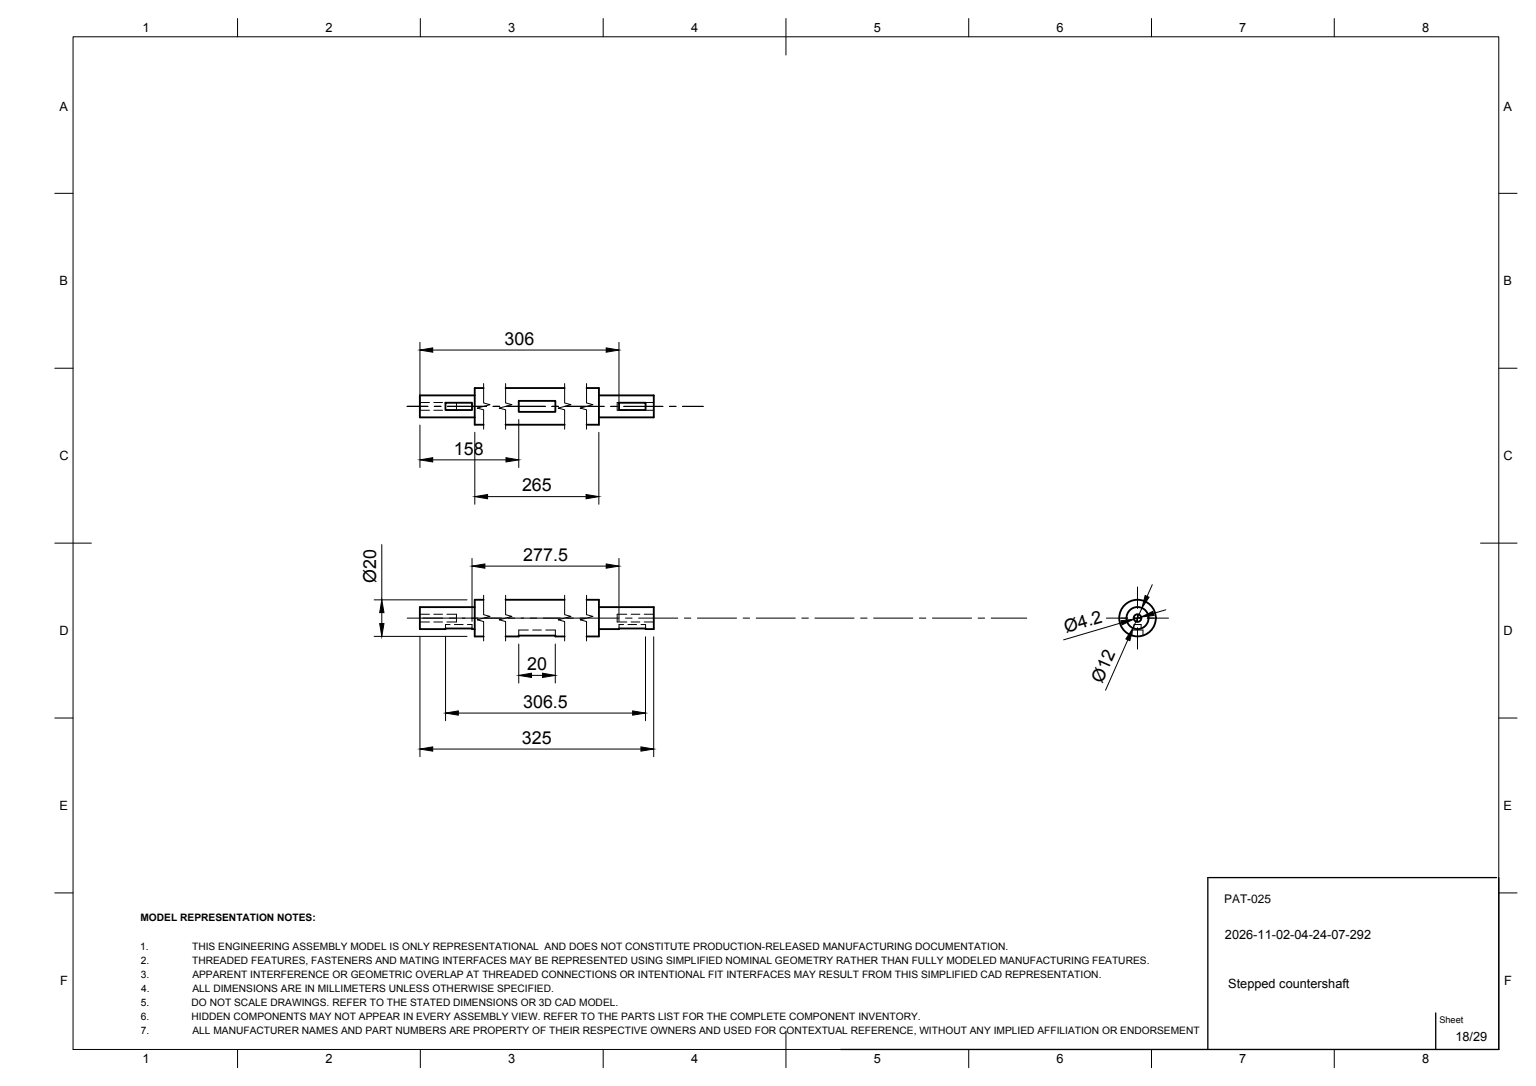
ISO-10303-21;
HEADER;
/* Generated by software containing ST-Developer
 * from STEP Tools, Inc. (www.steptools.com) 
 */

FILE_DESCRIPTION(
/* description */ ('Counter shaft with two pulleys and keyed hub'),
/* implementation_level */ '2;1');

FILE_NAME(
/* name */ 'Stepped countershaft.step',
/* time_stamp */ '2026-10-27T10:46:10-07:00',
/* author */ (''),
/* organization */ (''),
/* preprocessor_version */ 'ST-DEVELOPER v20.2',
/* originating_system */ 'Autodesk Translation Framework v15.17.0.0',
/* authorisation */ '');

FILE_SCHEMA (('AUTOMOTIVE_DESIGN { 1 0 10303 214 3 1 1 }'));
ENDSEC;

DATA;
#10=MECHANICAL_DESIGN_GEOMETRIC_PRESENTATION_REPRESENTATION('',(#302),#10821);
#251=SHAPE_REPRESENTATION_RELATIONSHIP('SRR','None',#10939,#276);
#276=ADVANCED_BREP_SHAPE_REPRESENTATION('',(#327),#10807);
#302=STYLED_ITEM('',(#11135),#327);
#327=MANIFOLD_SOLID_BREP('Body1',#5586);
#388=FACE_BOUND('',#1069,.T.);
#389=FACE_BOUND('',#1071,.T.);
#390=FACE_BOUND('',#1073,.T.);
#391=FACE_BOUND('',#1075,.T.);
#392=FACE_BOUND('',#1077,.T.);
#393=FACE_BOUND('',#1079,.T.);
#394=FACE_BOUND('',#1081,.T.);
#494=PLANE('',#6072);
#495=PLANE('',#6073);
#496=PLANE('',#6075);
#497=PLANE('',#6076);
#498=PLANE('',#6077);
#499=PLANE('',#6082);
#500=PLANE('',#6086);
#501=PLANE('',#6087);
#502=PLANE('',#6088);
#503=PLANE('',#6090);
#504=PLANE('',#6091);
#505=PLANE('',#6092);
#506=PLANE('',#6094);
#507=PLANE('',#6095);
#508=PLANE('',#6097);
#509=PLANE('',#6098);
#510=PLANE('',#6099);
#511=PLANE('',#6104);
#512=PLANE('',#6108);
#513=PLANE('',#6112);
#514=PLANE('',#6113);
#687=FACE_OUTER_BOUND('',#1049,.T.);
#688=FACE_OUTER_BOUND('',#1050,.T.);
#689=FACE_OUTER_BOUND('',#1051,.T.);
#690=FACE_OUTER_BOUND('',#1052,.T.);
#691=FACE_OUTER_BOUND('',#1053,.T.);
#692=FACE_OUTER_BOUND('',#1054,.T.);
#693=FACE_OUTER_BOUND('',#1055,.T.);
#694=FACE_OUTER_BOUND('',#1056,.T.);
#695=FACE_OUTER_BOUND('',#1057,.T.);
#696=FACE_OUTER_BOUND('',#1058,.T.);
#697=FACE_OUTER_BOUND('',#1059,.T.);
#698=FACE_OUTER_BOUND('',#1060,.T.);
#699=FACE_OUTER_BOUND('',#1061,.T.);
#700=FACE_OUTER_BOUND('',#1062,.T.);
#701=FACE_OUTER_BOUND('',#1063,.T.);
#702=FACE_OUTER_BOUND('',#1064,.T.);
#703=FACE_OUTER_BOUND('',#1065,.T.);
#704=FACE_OUTER_BOUND('',#1066,.T.);
#705=FACE_OUTER_BOUND('',#1067,.T.);
#706=FACE_OUTER_BOUND('',#1068,.T.);
#707=FACE_OUTER_BOUND('',#1070,.T.);
#708=FACE_OUTER_BOUND('',#1072,.T.);
#709=FACE_OUTER_BOUND('',#1074,.T.);
#710=FACE_OUTER_BOUND('',#1076,.T.);
#711=FACE_OUTER_BOUND('',#1078,.T.);
#712=FACE_OUTER_BOUND('',#1080,.T.);
#1049=EDGE_LOOP('',(#4057,#4058,#4059,#4060));
#1050=EDGE_LOOP('',(#4061,#4062,#4063,#4064));
#1051=EDGE_LOOP('',(#4065,#4066,#4067,#4068));
#1052=EDGE_LOOP('',(#4069,#4070,#4071,#4072));
#1053=EDGE_LOOP('',(#4073,#4074,#4075,#4076));
#1054=EDGE_LOOP('',(#4077,#4078,#4079,#4080));
#1055=EDGE_LOOP('',(#4081));
#1056=EDGE_LOOP('',(#4082,#4083,#4084,#4085));
#1057=EDGE_LOOP('',(#4086));
#1058=EDGE_LOOP('',(#4087,#4088,#4089,#4090));
#1059=EDGE_LOOP('',(#4091,#4092,#4093,#4094));
#1060=EDGE_LOOP('',(#4095,#4096,#4097,#4098));
#1061=EDGE_LOOP('',(#4099,#4100,#4101,#4102));
#1062=EDGE_LOOP('',(#4103,#4104,#4105,#4106));
#1063=EDGE_LOOP('',(#4107,#4108,#4109,#4110));
#1064=EDGE_LOOP('',(#4111,#4112,#4113,#4114));
#1065=EDGE_LOOP('',(#4115,#4116,#4117,#4118));
#1066=EDGE_LOOP('',(#4119,#4120,#4121,#4122));
#1067=EDGE_LOOP('',(#4123,#4124,#4125,#4126));
#1068=EDGE_LOOP('',(#4127,#4128,#4129,#4130));
#1069=EDGE_LOOP('',(#4131,#4132,#4133,#4134));
#1070=EDGE_LOOP('',(#4135));
#1071=EDGE_LOOP('',(#4136));
#1072=EDGE_LOOP('',(#4137,#4138,#4139,#4140));
#1073=EDGE_LOOP('',(#4141,#4142,#4143,#4144));
#1074=EDGE_LOOP('',(#4145));
#1075=EDGE_LOOP('',(#4146));
#1076=EDGE_LOOP('',(#4147,#4148,#4149,#4150));
#1077=EDGE_LOOP('',(#4151,#4152,#4153,#4154));
#1078=EDGE_LOOP('',(#4155));
#1079=EDGE_LOOP('',(#4156));
#1080=EDGE_LOOP('',(#4157));
#1081=EDGE_LOOP('',(#4158));
#1436=LINE('',#9220,#1825);
#1437=LINE('',#9222,#1826);
#1438=LINE('',#9224,#1827);
#1439=LINE('',#9225,#1828);
#1440=LINE('',#9230,#1829);
#1441=LINE('',#9231,#1830);
#1442=LINE('',#9234,#1831);
#1443=LINE('',#9236,#1832);
#1444=LINE('',#9237,#1833);
#1445=LINE('',#9239,#1834);
#1446=LINE('',#9246,#1835);
#1447=LINE('',#9253,#1836);
#1448=LINE('',#9259,#1837);
#1449=LINE('',#9261,#1838);
#1450=LINE('',#9263,#1839);
#1451=LINE('',#9264,#1840);
#1452=LINE('',#9269,#1841);
#1453=LINE('',#9270,#1842);
#1454=LINE('',#9273,#1843);
#1455=LINE('',#9275,#1844);
#1456=LINE('',#9276,#1845);
#1457=LINE('',#9278,#1846);
#1458=LINE('',#9284,#1847);
#1459=LINE('',#9286,#1848);
#1460=LINE('',#9288,#1849);
#1461=LINE('',#9289,#1850);
#1462=LINE('',#9294,#1851);
#1463=LINE('',#9295,#1852);
#1464=LINE('',#9298,#1853);
#1465=LINE('',#9300,#1854);
#1466=LINE('',#9301,#1855);
#1467=LINE('',#9303,#1856);
#1468=LINE('',#9310,#1857);
#1469=LINE('',#9317,#1858);
#1470=LINE('',#9324,#1859);
#1825=VECTOR('',#7080,1.);
#1826=VECTOR('',#7081,1.);
#1827=VECTOR('',#7082,1.);
#1828=VECTOR('',#7083,1.);
#1829=VECTOR('',#7088,1.);
#1830=VECTOR('',#7089,1.);
#1831=VECTOR('',#7092,1.);
#1832=VECTOR('',#7093,1.);
#1833=VECTOR('',#7094,1.);
#1834=VECTOR('',#7097,1.);
#1835=VECTOR('',#7106,0.21);
#1836=VECTOR('',#7115,0.21);
#1837=VECTOR('',#7122,1.);
#1838=VECTOR('',#7123,1.);
#1839=VECTOR('',#7124,1.);
#1840=VECTOR('',#7125,1.);
#1841=VECTOR('',#7130,1.);
#1842=VECTOR('',#7131,1.);
#1843=VECTOR('',#7134,1.);
#1844=VECTOR('',#7135,1.);
#1845=VECTOR('',#7136,1.);
#1846=VECTOR('',#7139,1.);
#1847=VECTOR('',#7146,1.);
#1848=VECTOR('',#7147,1.);
#1849=VECTOR('',#7148,1.);
#1850=VECTOR('',#7149,1.);
#1851=VECTOR('',#7154,1.);
#1852=VECTOR('',#7155,1.);
#1853=VECTOR('',#7158,1.);
#1854=VECTOR('',#7159,1.);
#1855=VECTOR('',#7160,1.);
#1856=VECTOR('',#7163,1.);
#1857=VECTOR('',#7172,0.6);
#1858=VECTOR('',#7181,0.6);
#1859=VECTOR('',#7190,1.);
#2146=CIRCLE('',#6074,1.);
#2147=CIRCLE('',#6078,1.);
#2148=CIRCLE('',#6080,0.21);
#2149=CIRCLE('',#6081,0.21);
#2150=CIRCLE('',#6084,0.21);
#2151=CIRCLE('',#6085,0.21);
#2152=CIRCLE('',#6089,0.6);
#2153=CIRCLE('',#6093,0.6);
#2154=CIRCLE('',#6096,0.6);
#2155=CIRCLE('',#6100,0.6);
#2156=CIRCLE('',#6102,0.6);
#2157=CIRCLE('',#6103,0.6);
#2158=CIRCLE('',#6106,0.6);
#2159=CIRCLE('',#6107,0.6);
#2160=CIRCLE('',#6110,1.);
#2161=CIRCLE('',#6111,1.);
#2533=VERTEX_POINT('',#9218);
#2534=VERTEX_POINT('',#9219);
#2535=VERTEX_POINT('',#9221);
#2536=VERTEX_POINT('',#9223);
#2537=VERTEX_POINT('',#9227);
#2538=VERTEX_POINT('',#9229);
#2539=VERTEX_POINT('',#9233);
#2540=VERTEX_POINT('',#9235);
#2541=VERTEX_POINT('',#9243);
#2542=VERTEX_POINT('',#9245);
#2543=VERTEX_POINT('',#9250);
#2544=VERTEX_POINT('',#9252);
#2545=VERTEX_POINT('',#9257);
#2546=VERTEX_POINT('',#9258);
#2547=VERTEX_POINT('',#9260);
#2548=VERTEX_POINT('',#9262);
#2549=VERTEX_POINT('',#9266);
#2550=VERTEX_POINT('',#9268);
#2551=VERTEX_POINT('',#9272);
#2552=VERTEX_POINT('',#9274);
#2553=VERTEX_POINT('',#9282);
#2554=VERTEX_POINT('',#9283);
#2555=VERTEX_POINT('',#9285);
#2556=VERTEX_POINT('',#9287);
#2557=VERTEX_POINT('',#9291);
#2558=VERTEX_POINT('',#9293);
#2559=VERTEX_POINT('',#9297);
#2560=VERTEX_POINT('',#9299);
#2561=VERTEX_POINT('',#9307);
#2562=VERTEX_POINT('',#9309);
#2563=VERTEX_POINT('',#9314);
#2564=VERTEX_POINT('',#9316);
#2565=VERTEX_POINT('',#9321);
#2566=VERTEX_POINT('',#9323);
#3101=EDGE_CURVE('',#2533,#2534,#1436,.T.);
#3102=EDGE_CURVE('',#2533,#2535,#1437,.T.);
#3103=EDGE_CURVE('',#2536,#2535,#1438,.T.);
#3104=EDGE_CURVE('',#2536,#2534,#1439,.T.);
#3105=EDGE_CURVE('',#2534,#2537,#2146,.T.);
#3106=EDGE_CURVE('',#2538,#2536,#1440,.T.);
#3107=EDGE_CURVE('',#2537,#2538,#1441,.T.);
#3108=EDGE_CURVE('',#2537,#2539,#1442,.T.);
#3109=EDGE_CURVE('',#2538,#2540,#1443,.T.);
#3110=EDGE_CURVE('',#2540,#2539,#1444,.T.);
#3111=EDGE_CURVE('',#2535,#2540,#1445,.T.);
#3112=EDGE_CURVE('',#2539,#2533,#2147,.T.);
#3113=EDGE_CURVE('',#2541,#2541,#2148,.T.);
#3114=EDGE_CURVE('',#2541,#2542,#1446,.T.);
#3115=EDGE_CURVE('',#2542,#2542,#2149,.T.);
#3116=EDGE_CURVE('',#2543,#2543,#2150,.T.);
#3117=EDGE_CURVE('',#2543,#2544,#1447,.T.);
#3118=EDGE_CURVE('',#2544,#2544,#2151,.T.);
#3119=EDGE_CURVE('',#2545,#2546,#1448,.T.);
#3120=EDGE_CURVE('',#2545,#2547,#1449,.T.);
#3121=EDGE_CURVE('',#2548,#2547,#1450,.T.);
#3122=EDGE_CURVE('',#2548,#2546,#1451,.T.);
#3123=EDGE_CURVE('',#2546,#2549,#2152,.T.);
#3124=EDGE_CURVE('',#2550,#2548,#1452,.T.);
#3125=EDGE_CURVE('',#2549,#2550,#1453,.T.);
#3126=EDGE_CURVE('',#2549,#2551,#1454,.T.);
#3127=EDGE_CURVE('',#2550,#2552,#1455,.T.);
#3128=EDGE_CURVE('',#2552,#2551,#1456,.T.);
#3129=EDGE_CURVE('',#2547,#2552,#1457,.T.);
#3130=EDGE_CURVE('',#2551,#2545,#2153,.T.);
#3131=EDGE_CURVE('',#2553,#2554,#1458,.T.);
#3132=EDGE_CURVE('',#2553,#2555,#1459,.T.);
#3133=EDGE_CURVE('',#2556,#2555,#1460,.T.);
#3134=EDGE_CURVE('',#2556,#2554,#1461,.T.);
#3135=EDGE_CURVE('',#2554,#2557,#2154,.T.);
#3136=EDGE_CURVE('',#2558,#2556,#1462,.T.);
#3137=EDGE_CURVE('',#2557,#2558,#1463,.T.);
#3138=EDGE_CURVE('',#2557,#2559,#1464,.T.);
#3139=EDGE_CURVE('',#2558,#2560,#1465,.T.);
#3140=EDGE_CURVE('',#2560,#2559,#1466,.T.);
#3141=EDGE_CURVE('',#2555,#2560,#1467,.T.);
#3142=EDGE_CURVE('',#2559,#2553,#2155,.T.);
#3143=EDGE_CURVE('',#2561,#2561,#2156,.T.);
#3144=EDGE_CURVE('',#2561,#2562,#1468,.T.);
#3145=EDGE_CURVE('',#2562,#2562,#2157,.T.);
#3146=EDGE_CURVE('',#2563,#2563,#2158,.T.);
#3147=EDGE_CURVE('',#2563,#2564,#1469,.T.);
#3148=EDGE_CURVE('',#2564,#2564,#2159,.T.);
#3149=EDGE_CURVE('',#2565,#2565,#2160,.T.);
#3150=EDGE_CURVE('',#2565,#2566,#1470,.T.);
#3151=EDGE_CURVE('',#2566,#2566,#2161,.T.);
#4057=ORIENTED_EDGE('',*,*,#3101,.F.);
#4058=ORIENTED_EDGE('',*,*,#3102,.T.);
#4059=ORIENTED_EDGE('',*,*,#3103,.F.);
#4060=ORIENTED_EDGE('',*,*,#3104,.T.);
#4061=ORIENTED_EDGE('',*,*,#3105,.F.);
#4062=ORIENTED_EDGE('',*,*,#3104,.F.);
#4063=ORIENTED_EDGE('',*,*,#3106,.F.);
#4064=ORIENTED_EDGE('',*,*,#3107,.F.);
#4065=ORIENTED_EDGE('',*,*,#3108,.F.);
#4066=ORIENTED_EDGE('',*,*,#3107,.T.);
#4067=ORIENTED_EDGE('',*,*,#3109,.T.);
#4068=ORIENTED_EDGE('',*,*,#3110,.T.);
#4069=ORIENTED_EDGE('',*,*,#3106,.T.);
#4070=ORIENTED_EDGE('',*,*,#3103,.T.);
#4071=ORIENTED_EDGE('',*,*,#3111,.T.);
#4072=ORIENTED_EDGE('',*,*,#3109,.F.);
#4073=ORIENTED_EDGE('',*,*,#3112,.F.);
#4074=ORIENTED_EDGE('',*,*,#3110,.F.);
#4075=ORIENTED_EDGE('',*,*,#3111,.F.);
#4076=ORIENTED_EDGE('',*,*,#3102,.F.);
#4077=ORIENTED_EDGE('',*,*,#3113,.F.);
#4078=ORIENTED_EDGE('',*,*,#3114,.T.);
#4079=ORIENTED_EDGE('',*,*,#3115,.F.);
#4080=ORIENTED_EDGE('',*,*,#3114,.F.);
#4081=ORIENTED_EDGE('',*,*,#3113,.T.);
#4082=ORIENTED_EDGE('',*,*,#3116,.F.);
#4083=ORIENTED_EDGE('',*,*,#3117,.T.);
#4084=ORIENTED_EDGE('',*,*,#3118,.T.);
#4085=ORIENTED_EDGE('',*,*,#3117,.F.);
#4086=ORIENTED_EDGE('',*,*,#3118,.F.);
#4087=ORIENTED_EDGE('',*,*,#3119,.F.);
#4088=ORIENTED_EDGE('',*,*,#3120,.T.);
#4089=ORIENTED_EDGE('',*,*,#3121,.F.);
#4090=ORIENTED_EDGE('',*,*,#3122,.T.);
#4091=ORIENTED_EDGE('',*,*,#3123,.F.);
#4092=ORIENTED_EDGE('',*,*,#3122,.F.);
#4093=ORIENTED_EDGE('',*,*,#3124,.F.);
#4094=ORIENTED_EDGE('',*,*,#3125,.F.);
#4095=ORIENTED_EDGE('',*,*,#3126,.F.);
#4096=ORIENTED_EDGE('',*,*,#3125,.T.);
#4097=ORIENTED_EDGE('',*,*,#3127,.T.);
#4098=ORIENTED_EDGE('',*,*,#3128,.T.);
#4099=ORIENTED_EDGE('',*,*,#3124,.T.);
#4100=ORIENTED_EDGE('',*,*,#3121,.T.);
#4101=ORIENTED_EDGE('',*,*,#3129,.T.);
#4102=ORIENTED_EDGE('',*,*,#3127,.F.);
#4103=ORIENTED_EDGE('',*,*,#3130,.F.);
#4104=ORIENTED_EDGE('',*,*,#3128,.F.);
#4105=ORIENTED_EDGE('',*,*,#3129,.F.);
#4106=ORIENTED_EDGE('',*,*,#3120,.F.);
#4107=ORIENTED_EDGE('',*,*,#3131,.F.);
#4108=ORIENTED_EDGE('',*,*,#3132,.T.);
#4109=ORIENTED_EDGE('',*,*,#3133,.F.);
#4110=ORIENTED_EDGE('',*,*,#3134,.T.);
#4111=ORIENTED_EDGE('',*,*,#3135,.F.);
#4112=ORIENTED_EDGE('',*,*,#3134,.F.);
#4113=ORIENTED_EDGE('',*,*,#3136,.F.);
#4114=ORIENTED_EDGE('',*,*,#3137,.F.);
#4115=ORIENTED_EDGE('',*,*,#3138,.F.);
#4116=ORIENTED_EDGE('',*,*,#3137,.T.);
#4117=ORIENTED_EDGE('',*,*,#3139,.T.);
#4118=ORIENTED_EDGE('',*,*,#3140,.T.);
#4119=ORIENTED_EDGE('',*,*,#3136,.T.);
#4120=ORIENTED_EDGE('',*,*,#3133,.T.);
#4121=ORIENTED_EDGE('',*,*,#3141,.T.);
#4122=ORIENTED_EDGE('',*,*,#3139,.F.);
#4123=ORIENTED_EDGE('',*,*,#3142,.F.);
#4124=ORIENTED_EDGE('',*,*,#3140,.F.);
#4125=ORIENTED_EDGE('',*,*,#3141,.F.);
#4126=ORIENTED_EDGE('',*,*,#3132,.F.);
#4127=ORIENTED_EDGE('',*,*,#3143,.F.);
#4128=ORIENTED_EDGE('',*,*,#3144,.T.);
#4129=ORIENTED_EDGE('',*,*,#3145,.F.);
#4130=ORIENTED_EDGE('',*,*,#3144,.F.);
#4131=ORIENTED_EDGE('',*,*,#3126,.T.);
#4132=ORIENTED_EDGE('',*,*,#3130,.T.);
#4133=ORIENTED_EDGE('',*,*,#3119,.T.);
#4134=ORIENTED_EDGE('',*,*,#3123,.T.);
#4135=ORIENTED_EDGE('',*,*,#3143,.T.);
#4136=ORIENTED_EDGE('',*,*,#3115,.T.);
#4137=ORIENTED_EDGE('',*,*,#3146,.F.);
#4138=ORIENTED_EDGE('',*,*,#3147,.T.);
#4139=ORIENTED_EDGE('',*,*,#3148,.T.);
#4140=ORIENTED_EDGE('',*,*,#3147,.F.);
#4141=ORIENTED_EDGE('',*,*,#3138,.T.);
#4142=ORIENTED_EDGE('',*,*,#3142,.T.);
#4143=ORIENTED_EDGE('',*,*,#3131,.T.);
#4144=ORIENTED_EDGE('',*,*,#3135,.T.);
#4145=ORIENTED_EDGE('',*,*,#3148,.F.);
#4146=ORIENTED_EDGE('',*,*,#3116,.T.);
#4147=ORIENTED_EDGE('',*,*,#3149,.F.);
#4148=ORIENTED_EDGE('',*,*,#3150,.T.);
#4149=ORIENTED_EDGE('',*,*,#3151,.T.);
#4150=ORIENTED_EDGE('',*,*,#3150,.F.);
#4151=ORIENTED_EDGE('',*,*,#3108,.T.);
#4152=ORIENTED_EDGE('',*,*,#3112,.T.);
#4153=ORIENTED_EDGE('',*,*,#3101,.T.);
#4154=ORIENTED_EDGE('',*,*,#3105,.T.);
#4155=ORIENTED_EDGE('',*,*,#3149,.T.);
#4156=ORIENTED_EDGE('',*,*,#3145,.T.);
#4157=ORIENTED_EDGE('',*,*,#3151,.F.);
#4158=ORIENTED_EDGE('',*,*,#3146,.T.);
#5144=CYLINDRICAL_SURFACE('',#6079,0.21);
#5145=CYLINDRICAL_SURFACE('',#6083,0.21);
#5146=CYLINDRICAL_SURFACE('',#6101,0.6);
#5147=CYLINDRICAL_SURFACE('',#6105,0.6);
#5148=CYLINDRICAL_SURFACE('',#6109,1.);
#5358=ADVANCED_FACE('',(#687),#494,.F.);
#5359=ADVANCED_FACE('',(#688),#495,.T.);
#5360=ADVANCED_FACE('',(#689),#496,.F.);
#5361=ADVANCED_FACE('',(#690),#497,.F.);
#5362=ADVANCED_FACE('',(#691),#498,.F.);
#5363=ADVANCED_FACE('',(#692),#5144,.F.);
#5364=ADVANCED_FACE('',(#693),#499,.T.);
#5365=ADVANCED_FACE('',(#694),#5145,.F.);
#5366=ADVANCED_FACE('',(#695),#500,.F.);
#5367=ADVANCED_FACE('',(#696),#501,.F.);
#5368=ADVANCED_FACE('',(#697),#502,.T.);
#5369=ADVANCED_FACE('',(#698),#503,.F.);
#5370=ADVANCED_FACE('',(#699),#504,.F.);
#5371=ADVANCED_FACE('',(#700),#505,.F.);
#5372=ADVANCED_FACE('',(#701),#506,.F.);
#5373=ADVANCED_FACE('',(#702),#507,.T.);
#5374=ADVANCED_FACE('',(#703),#508,.F.);
#5375=ADVANCED_FACE('',(#704),#509,.F.);
#5376=ADVANCED_FACE('',(#705),#510,.F.);
#5377=ADVANCED_FACE('',(#706,#388),#5146,.T.);
#5378=ADVANCED_FACE('',(#707,#389),#511,.T.);
#5379=ADVANCED_FACE('',(#708,#390),#5147,.T.);
#5380=ADVANCED_FACE('',(#709,#391),#512,.F.);
#5381=ADVANCED_FACE('',(#710,#392),#5148,.T.);
#5382=ADVANCED_FACE('',(#711,#393),#513,.T.);
#5383=ADVANCED_FACE('',(#712,#394),#514,.F.);
#5586=CLOSED_SHELL('',(#5358,#5359,#5360,#5361,#5362,#5363,#5364,#5365,
#5366,#5367,#5368,#5369,#5370,#5371,#5372,#5373,#5374,#5375,#5376,#5377,
#5378,#5379,#5380,#5381,#5382,#5383));
#6071=AXIS2_PLACEMENT_3D('',#9216,#7076,#7077);
#6072=AXIS2_PLACEMENT_3D('',#9217,#7078,#7079);
#6073=AXIS2_PLACEMENT_3D('',#9226,#7084,#7085);
#6074=AXIS2_PLACEMENT_3D('',#9228,#7086,#7087);
#6075=AXIS2_PLACEMENT_3D('',#9232,#7090,#7091);
#6076=AXIS2_PLACEMENT_3D('',#9238,#7095,#7096);
#6077=AXIS2_PLACEMENT_3D('',#9240,#7098,#7099);
#6078=AXIS2_PLACEMENT_3D('',#9241,#7100,#7101);
#6079=AXIS2_PLACEMENT_3D('',#9242,#7102,#7103);
#6080=AXIS2_PLACEMENT_3D('',#9244,#7104,#7105);
#6081=AXIS2_PLACEMENT_3D('',#9247,#7107,#7108);
#6082=AXIS2_PLACEMENT_3D('',#9248,#7109,#7110);
#6083=AXIS2_PLACEMENT_3D('',#9249,#7111,#7112);
#6084=AXIS2_PLACEMENT_3D('',#9251,#7113,#7114);
#6085=AXIS2_PLACEMENT_3D('',#9254,#7116,#7117);
#6086=AXIS2_PLACEMENT_3D('',#9255,#7118,#7119);
#6087=AXIS2_PLACEMENT_3D('',#9256,#7120,#7121);
#6088=AXIS2_PLACEMENT_3D('',#9265,#7126,#7127);
#6089=AXIS2_PLACEMENT_3D('',#9267,#7128,#7129);
#6090=AXIS2_PLACEMENT_3D('',#9271,#7132,#7133);
#6091=AXIS2_PLACEMENT_3D('',#9277,#7137,#7138);
#6092=AXIS2_PLACEMENT_3D('',#9279,#7140,#7141);
#6093=AXIS2_PLACEMENT_3D('',#9280,#7142,#7143);
#6094=AXIS2_PLACEMENT_3D('',#9281,#7144,#7145);
#6095=AXIS2_PLACEMENT_3D('',#9290,#7150,#7151);
#6096=AXIS2_PLACEMENT_3D('',#9292,#7152,#7153);
#6097=AXIS2_PLACEMENT_3D('',#9296,#7156,#7157);
#6098=AXIS2_PLACEMENT_3D('',#9302,#7161,#7162);
#6099=AXIS2_PLACEMENT_3D('',#9304,#7164,#7165);
#6100=AXIS2_PLACEMENT_3D('',#9305,#7166,#7167);
#6101=AXIS2_PLACEMENT_3D('',#9306,#7168,#7169);
#6102=AXIS2_PLACEMENT_3D('',#9308,#7170,#7171);
#6103=AXIS2_PLACEMENT_3D('',#9311,#7173,#7174);
#6104=AXIS2_PLACEMENT_3D('',#9312,#7175,#7176);
#6105=AXIS2_PLACEMENT_3D('',#9313,#7177,#7178);
#6106=AXIS2_PLACEMENT_3D('',#9315,#7179,#7180);
#6107=AXIS2_PLACEMENT_3D('',#9318,#7182,#7183);
#6108=AXIS2_PLACEMENT_3D('',#9319,#7184,#7185);
#6109=AXIS2_PLACEMENT_3D('',#9320,#7186,#7187);
#6110=AXIS2_PLACEMENT_3D('',#9322,#7188,#7189);
#6111=AXIS2_PLACEMENT_3D('',#9325,#7191,#7192);
#6112=AXIS2_PLACEMENT_3D('',#9326,#7193,#7194);
#6113=AXIS2_PLACEMENT_3D('',#9327,#7195,#7196);
#7076=DIRECTION('axis',(0.,0.,1.));
#7077=DIRECTION('refdir',(1.,0.,0.));
#7078=DIRECTION('center_axis',(-1.,0.,0.));
#7079=DIRECTION('ref_axis',(0.,0.,1.));
#7080=DIRECTION('',(0.,-1.,0.));
#7081=DIRECTION('',(0.,0.,1.));
#7082=DIRECTION('',(0.,1.,0.));
#7083=DIRECTION('',(0.,0.,-1.));
#7084=DIRECTION('center_axis',(0.,1.,0.));
#7085=DIRECTION('ref_axis',(1.,0.,0.));
#7086=DIRECTION('center_axis',(0.,-1.,0.));
#7087=DIRECTION('ref_axis',(1.,0.,0.));
#7088=DIRECTION('',(-1.,0.,0.));
#7089=DIRECTION('',(0.,0.,1.));
#7090=DIRECTION('center_axis',(1.,0.,0.));
#7091=DIRECTION('ref_axis',(0.,0.,-1.));
#7092=DIRECTION('',(0.,1.,0.));
#7093=DIRECTION('',(0.,1.,0.));
#7094=DIRECTION('',(0.,0.,-1.));
#7095=DIRECTION('center_axis',(0.,0.,1.));
#7096=DIRECTION('ref_axis',(1.,0.,0.));
#7097=DIRECTION('',(1.,0.,0.));
#7098=DIRECTION('center_axis',(0.,1.,0.));
#7099=DIRECTION('ref_axis',(0.,0.,1.));
#7100=DIRECTION('center_axis',(0.,1.,0.));
#7101=DIRECTION('ref_axis',(1.,0.,0.));
#7102=DIRECTION('center_axis',(0.,1.,0.));
#7103=DIRECTION('ref_axis',(1.,0.,0.));
#7104=DIRECTION('center_axis',(0.,1.,0.));
#7105=DIRECTION('ref_axis',(1.,0.,0.));
#7106=DIRECTION('',(0.,1.,0.));
#7107=DIRECTION('center_axis',(0.,-1.,0.));
#7108=DIRECTION('ref_axis',(1.,0.,0.));
#7109=DIRECTION('center_axis',(0.,1.,0.));
#7110=DIRECTION('ref_axis',(1.,0.,0.));
#7111=DIRECTION('center_axis',(0.,1.,0.));
#7112=DIRECTION('ref_axis',(1.,0.,0.));
#7113=DIRECTION('center_axis',(0.,1.,0.));
#7114=DIRECTION('ref_axis',(1.,0.,0.));
#7115=DIRECTION('',(0.,1.,0.));
#7116=DIRECTION('center_axis',(0.,1.,0.));
#7117=DIRECTION('ref_axis',(1.,0.,0.));
#7118=DIRECTION('center_axis',(0.,1.,0.));
#7119=DIRECTION('ref_axis',(1.,0.,0.));
#7120=DIRECTION('center_axis',(-1.,0.,0.));
#7121=DIRECTION('ref_axis',(0.,0.,1.));
#7122=DIRECTION('',(0.,-1.,0.));
#7123=DIRECTION('',(0.,0.,1.));
#7124=DIRECTION('',(0.,1.,0.));
#7125=DIRECTION('',(0.,0.,-1.));
#7126=DIRECTION('center_axis',(0.,1.,0.));
#7127=DIRECTION('ref_axis',(1.,0.,0.));
#7128=DIRECTION('center_axis',(0.,-1.,0.));
#7129=DIRECTION('ref_axis',(1.,0.,0.));
#7130=DIRECTION('',(-1.,0.,0.));
#7131=DIRECTION('',(0.,0.,1.));
#7132=DIRECTION('center_axis',(1.,0.,0.));
#7133=DIRECTION('ref_axis',(0.,0.,-1.));
#7134=DIRECTION('',(0.,1.,0.));
#7135=DIRECTION('',(0.,1.,0.));
#7136=DIRECTION('',(0.,0.,-1.));
#7137=DIRECTION('center_axis',(0.,0.,1.));
#7138=DIRECTION('ref_axis',(1.,0.,0.));
#7139=DIRECTION('',(1.,0.,0.));
#7140=DIRECTION('center_axis',(0.,1.,0.));
#7141=DIRECTION('ref_axis',(0.,0.,1.));
#7142=DIRECTION('center_axis',(0.,1.,0.));
#7143=DIRECTION('ref_axis',(1.,0.,0.));
#7144=DIRECTION('center_axis',(-1.,0.,0.));
#7145=DIRECTION('ref_axis',(0.,0.,1.));
#7146=DIRECTION('',(0.,-1.,0.));
#7147=DIRECTION('',(0.,0.,1.));
#7148=DIRECTION('',(0.,1.,0.));
#7149=DIRECTION('',(0.,0.,-1.));
#7150=DIRECTION('center_axis',(0.,1.,0.));
#7151=DIRECTION('ref_axis',(1.,0.,0.));
#7152=DIRECTION('center_axis',(0.,-1.,0.));
#7153=DIRECTION('ref_axis',(1.,0.,0.));
#7154=DIRECTION('',(-1.,0.,0.));
#7155=DIRECTION('',(0.,0.,1.));
#7156=DIRECTION('center_axis',(1.,0.,0.));
#7157=DIRECTION('ref_axis',(0.,0.,-1.));
#7158=DIRECTION('',(0.,1.,0.));
#7159=DIRECTION('',(0.,1.,0.));
#7160=DIRECTION('',(0.,0.,-1.));
#7161=DIRECTION('center_axis',(0.,0.,1.));
#7162=DIRECTION('ref_axis',(1.,0.,0.));
#7163=DIRECTION('',(1.,0.,0.));
#7164=DIRECTION('center_axis',(0.,1.,0.));
#7165=DIRECTION('ref_axis',(0.,0.,1.));
#7166=DIRECTION('center_axis',(0.,1.,0.));
#7167=DIRECTION('ref_axis',(1.,0.,0.));
#7168=DIRECTION('center_axis',(0.,1.,0.));
#7169=DIRECTION('ref_axis',(1.,0.,0.));
#7170=DIRECTION('center_axis',(0.,1.,0.));
#7171=DIRECTION('ref_axis',(1.,0.,0.));
#7172=DIRECTION('',(0.,-1.,0.));
#7173=DIRECTION('center_axis',(0.,-1.,0.));
#7174=DIRECTION('ref_axis',(1.,0.,0.));
#7175=DIRECTION('center_axis',(0.,1.,0.));
#7176=DIRECTION('ref_axis',(1.,0.,0.));
#7177=DIRECTION('center_axis',(0.,1.,0.));
#7178=DIRECTION('ref_axis',(1.,0.,0.));
#7179=DIRECTION('center_axis',(0.,1.,0.));
#7180=DIRECTION('ref_axis',(1.,0.,0.));
#7181=DIRECTION('',(0.,-1.,0.));
#7182=DIRECTION('center_axis',(0.,1.,0.));
#7183=DIRECTION('ref_axis',(1.,0.,0.));
#7184=DIRECTION('center_axis',(0.,1.,0.));
#7185=DIRECTION('ref_axis',(1.,0.,0.));
#7186=DIRECTION('center_axis',(0.,1.,0.));
#7187=DIRECTION('ref_axis',(1.,0.,0.));
#7188=DIRECTION('center_axis',(0.,1.,0.));
#7189=DIRECTION('ref_axis',(1.,0.,0.));
#7190=DIRECTION('',(0.,-1.,0.));
#7191=DIRECTION('center_axis',(0.,1.,0.));
#7192=DIRECTION('ref_axis',(1.,0.,0.));
#7193=DIRECTION('center_axis',(0.,1.,0.));
#7194=DIRECTION('ref_axis',(1.,0.,0.));
#7195=DIRECTION('center_axis',(0.,1.,0.));
#7196=DIRECTION('ref_axis',(1.,0.,0.));
#9216=CARTESIAN_POINT('',(0.,0.,0.));
#9217=CARTESIAN_POINT('Origin',(-0.3,9.2,3.43));
#9218=CARTESIAN_POINT('',(-0.3,11.2,3.57606079858305));
#9219=CARTESIAN_POINT('',(-0.3,9.2,3.57606079858305));
#9220=CARTESIAN_POINT('',(-0.3,-2.5,3.57606079858305));
#9221=CARTESIAN_POINT('',(-0.3,11.2,3.88));
#9222=CARTESIAN_POINT('',(-0.3,11.2,3.88));
#9223=CARTESIAN_POINT('',(-0.3,9.2,3.88));
#9224=CARTESIAN_POINT('',(-0.3,9.2,3.88));
#9225=CARTESIAN_POINT('',(-0.3,9.2,3.88));
#9226=CARTESIAN_POINT('Origin',(0.,9.2,3.655));
#9227=CARTESIAN_POINT('',(0.3,9.2,3.57606079858305));
#9228=CARTESIAN_POINT('Origin',(0.,9.2,4.53));
#9229=CARTESIAN_POINT('',(0.3,9.2,3.88));
#9230=CARTESIAN_POINT('',(0.3,9.2,3.88));
#9231=CARTESIAN_POINT('',(0.3,9.2,3.43));
#9232=CARTESIAN_POINT('Origin',(0.3,9.2,3.88));
#9233=CARTESIAN_POINT('',(0.3,11.2,3.57606079858305));
#9234=CARTESIAN_POINT('',(0.3,-2.5,3.57606079858305));
#9235=CARTESIAN_POINT('',(0.3,11.2,3.88));
#9236=CARTESIAN_POINT('',(0.3,9.2,3.88));
#9237=CARTESIAN_POINT('',(0.3,11.2,3.43));
#9238=CARTESIAN_POINT('Origin',(-0.3,9.2,3.88));
#9239=CARTESIAN_POINT('',(0.3,11.2,3.88));
#9240=CARTESIAN_POINT('Origin',(0.,11.2,3.655));
#9241=CARTESIAN_POINT('Origin',(0.,11.2,4.53));
#9242=CARTESIAN_POINT('Origin',(0.,25.,4.53));
#9243=CARTESIAN_POINT('',(-0.21,25.,4.53));
#9244=CARTESIAN_POINT('Origin',(0.,25.,4.53));
#9245=CARTESIAN_POINT('',(-0.21,27.,4.53));
#9246=CARTESIAN_POINT('',(-0.21,25.,4.53));
#9247=CARTESIAN_POINT('Origin',(0.,27.,4.53));
#9248=CARTESIAN_POINT('Origin',(0.,25.,4.53));
#9249=CARTESIAN_POINT('Origin',(0.,-5.6,4.53));
#9250=CARTESIAN_POINT('',(-0.21,-5.5,4.53));
#9251=CARTESIAN_POINT('Origin',(0.,-5.5,4.53));
#9252=CARTESIAN_POINT('',(-0.21,-3.5,4.53));
#9253=CARTESIAN_POINT('',(-0.21,-5.6,4.53));
#9254=CARTESIAN_POINT('Origin',(0.,-3.5,4.53));
#9255=CARTESIAN_POINT('Origin',(0.,-3.5,4.53));
#9256=CARTESIAN_POINT('Origin',(-0.2,24.15,3.83));
#9257=CARTESIAN_POINT('',(-0.2,25.6,3.96431457505076));
#9258=CARTESIAN_POINT('',(-0.2,24.15,3.96431457505076));
#9259=CARTESIAN_POINT('',(-0.2,24.,3.96431457505076));
#9260=CARTESIAN_POINT('',(-0.2,25.6,4.18));
#9261=CARTESIAN_POINT('',(-0.2,25.6,4.18));
#9262=CARTESIAN_POINT('',(-0.2,24.15,4.18));
#9263=CARTESIAN_POINT('',(-0.2,24.15,4.18));
#9264=CARTESIAN_POINT('',(-0.2,24.15,4.18));
#9265=CARTESIAN_POINT('Origin',(0.,24.15,4.005));
#9266=CARTESIAN_POINT('',(0.2,24.15,3.96431457505076));
#9267=CARTESIAN_POINT('Origin',(0.,24.15,4.53));
#9268=CARTESIAN_POINT('',(0.2,24.15,4.18));
#9269=CARTESIAN_POINT('',(0.2,24.15,4.18));
#9270=CARTESIAN_POINT('',(0.2,24.15,3.83));
#9271=CARTESIAN_POINT('Origin',(0.2,24.15,4.18));
#9272=CARTESIAN_POINT('',(0.2,25.6,3.96431457505076));
#9273=CARTESIAN_POINT('',(0.2,24.,3.96431457505076));
#9274=CARTESIAN_POINT('',(0.2,25.6,4.18));
#9275=CARTESIAN_POINT('',(0.2,24.15,4.18));
#9276=CARTESIAN_POINT('',(0.2,25.6,3.83));
#9277=CARTESIAN_POINT('Origin',(-0.2,24.15,4.18));
#9278=CARTESIAN_POINT('',(0.2,25.6,4.18));
#9279=CARTESIAN_POINT('Origin',(0.,25.6,4.005));
#9280=CARTESIAN_POINT('Origin',(0.,25.6,4.53));
#9281=CARTESIAN_POINT('Origin',(-0.2,-5.05,3.83));
#9282=CARTESIAN_POINT('',(-0.2,-3.6,3.96431457505076));
#9283=CARTESIAN_POINT('',(-0.2,-5.05,3.96431457505076));
#9284=CARTESIAN_POINT('',(-0.2,-5.5,3.96431457505076));
#9285=CARTESIAN_POINT('',(-0.2,-3.6,4.18));
#9286=CARTESIAN_POINT('',(-0.2,-3.6,4.18));
#9287=CARTESIAN_POINT('',(-0.2,-5.05,4.18));
#9288=CARTESIAN_POINT('',(-0.2,-5.05,4.18));
#9289=CARTESIAN_POINT('',(-0.2,-5.05,4.18));
#9290=CARTESIAN_POINT('Origin',(0.,-5.05,4.005));
#9291=CARTESIAN_POINT('',(0.2,-5.05,3.96431457505076));
#9292=CARTESIAN_POINT('Origin',(0.,-5.05,4.53));
#9293=CARTESIAN_POINT('',(0.2,-5.05,4.18));
#9294=CARTESIAN_POINT('',(0.2,-5.05,4.18));
#9295=CARTESIAN_POINT('',(0.2,-5.05,3.83));
#9296=CARTESIAN_POINT('Origin',(0.2,-5.05,4.18));
#9297=CARTESIAN_POINT('',(0.2,-3.6,3.96431457505076));
#9298=CARTESIAN_POINT('',(0.2,-5.5,3.96431457505076));
#9299=CARTESIAN_POINT('',(0.2,-3.6,4.18));
#9300=CARTESIAN_POINT('',(0.2,-5.05,4.18));
#9301=CARTESIAN_POINT('',(0.2,-3.6,3.83));
#9302=CARTESIAN_POINT('Origin',(-0.2,-5.05,4.18));
#9303=CARTESIAN_POINT('',(0.2,-3.6,4.18));
#9304=CARTESIAN_POINT('Origin',(0.,-3.6,4.005));
#9305=CARTESIAN_POINT('Origin',(0.,-3.6,4.53));
#9306=CARTESIAN_POINT('Origin',(0.,24.,4.53));
#9307=CARTESIAN_POINT('',(-0.6,27.,4.53));
#9308=CARTESIAN_POINT('Origin',(0.,27.,4.53));
#9309=CARTESIAN_POINT('',(-0.6,24.,4.53));
#9310=CARTESIAN_POINT('',(-0.6,24.,4.53));
#9311=CARTESIAN_POINT('Origin',(0.,24.,4.53));
#9312=CARTESIAN_POINT('Origin',(0.,27.,4.53));
#9313=CARTESIAN_POINT('Origin',(0.,-5.5,4.53));
#9314=CARTESIAN_POINT('',(-0.6,-2.5,4.53));
#9315=CARTESIAN_POINT('Origin',(0.,-2.5,4.53));
#9316=CARTESIAN_POINT('',(-0.6,-5.5,4.53));
#9317=CARTESIAN_POINT('',(-0.6,-5.5,4.53));
#9318=CARTESIAN_POINT('Origin',(0.,-5.5,4.53));
#9319=CARTESIAN_POINT('Origin',(0.,-5.5,4.53));
#9320=CARTESIAN_POINT('Origin',(0.,-2.5,4.53));
#9321=CARTESIAN_POINT('',(-1.,24.,4.53));
#9322=CARTESIAN_POINT('Origin',(0.,24.,4.53));
#9323=CARTESIAN_POINT('',(-1.,-2.5,4.53));
#9324=CARTESIAN_POINT('',(-1.,-2.5,4.53));
#9325=CARTESIAN_POINT('Origin',(0.,-2.5,4.53));
#9326=CARTESIAN_POINT('Origin',(0.,24.,4.53));
#9327=CARTESIAN_POINT('Origin',(0.,-2.5,4.53));
#10777=UNCERTAINTY_MEASURE_WITH_UNIT(LENGTH_MEASURE(0.001),#10822,
'DISTANCE_ACCURACY_VALUE',
'Maximum model space distance between geometric entities at asserted c
onnectivities');
#10791=UNCERTAINTY_MEASURE_WITH_UNIT(LENGTH_MEASURE(0.001),#10822,
'DISTANCE_ACCURACY_VALUE',
'Maximum model space distance between geometric entities at asserted c
onnectivities');
#10807=(
GEOMETRIC_REPRESENTATION_CONTEXT(3)
GLOBAL_UNCERTAINTY_ASSIGNED_CONTEXT((#10777))
GLOBAL_UNIT_ASSIGNED_CONTEXT((#10822,#10824,#10825))
REPRESENTATION_CONTEXT('','3D')
);
#10821=(
GEOMETRIC_REPRESENTATION_CONTEXT(3)
GLOBAL_UNCERTAINTY_ASSIGNED_CONTEXT((#10791))
GLOBAL_UNIT_ASSIGNED_CONTEXT((#10822,#10824,#10825))
REPRESENTATION_CONTEXT('','3D')
);
#10822=(
LENGTH_UNIT()
NAMED_UNIT(*)
SI_UNIT(.CENTI.,.METRE.)
);
#10824=(
NAMED_UNIT(*)
PLANE_ANGLE_UNIT()
SI_UNIT($,.RADIAN.)
);
#10825=(
NAMED_UNIT(*)
SI_UNIT($,.STERADIAN.)
SOLID_ANGLE_UNIT()
);
#10841=SHAPE_DEFINITION_REPRESENTATION(#10889,#10939);
#10889=PRODUCT_DEFINITION_SHAPE('',$,#10969);
#10939=SHAPE_REPRESENTATION('',(#6071),#10807);
#10953=PRODUCT_DEFINITION_CONTEXT('part definition',#11042,'design');
#10969=PRODUCT_DEFINITION('Stepped countershaft','Stepped countershaft',
#10998,#10953);
#10998=PRODUCT_DEFINITION_FORMATION('',$,#11059);
#11042=APPLICATION_CONTEXT(
'Core Data for Automotive Mechanical Design Process');
#11043=PRODUCT_CONTEXT('part definition',#11042,'mechanical');
#11059=PRODUCT('Stepped countershaft','Stepped countershaft',
'Stepped countershaft',(#11043));
#11129=COLOUR_RGB('Grey',0.48,0.52,0.57);
#11130=FILL_AREA_STYLE_COLOUR('',#11129);
#11131=FILL_AREA_STYLE('',(#11130));
#11132=SURFACE_STYLE_FILL_AREA(#11131);
#11133=SURFACE_SIDE_STYLE('',(#11132));
#11134=SURFACE_STYLE_USAGE(.BOTH.,#11133);
#11135=PRESENTATION_STYLE_ASSIGNMENT((#11134));
ENDSEC;
END-ISO-10303-21;
